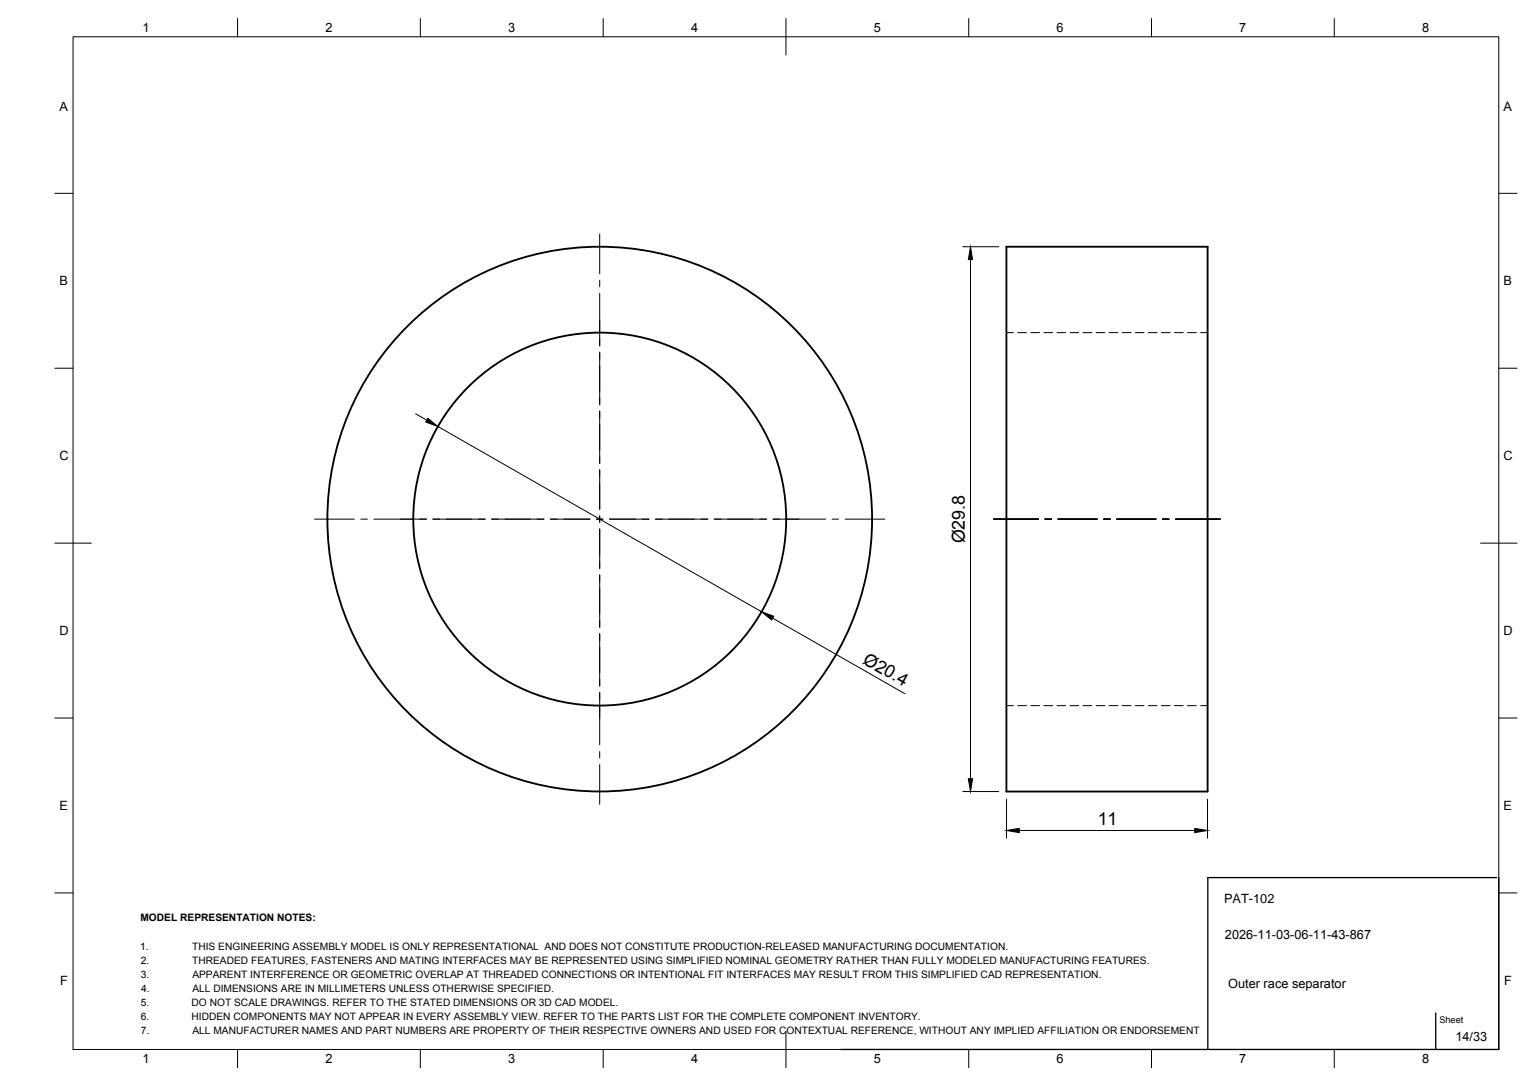
ISO-10303-21;
HEADER;
/* Generated by software containing ST-Developer
 * from STEP Tools, Inc. (www.steptools.com) 
 */

FILE_DESCRIPTION(
/* description */ ('Swing-away clamp arm'),
/* implementation_level */ '2;1');

FILE_NAME(
/* name */ 'Outer race separator.step',
/* time_stamp */ '2026-10-28T03:26:03-07:00',
/* author */ (''),
/* organization */ (''),
/* preprocessor_version */ 'ST-DEVELOPER v20.2',
/* originating_system */ 'Autodesk Translation Framework v15.17.0.0',
/* authorisation */ '');

FILE_SCHEMA (('AUTOMOTIVE_DESIGN { 1 0 10303 214 3 1 1 }'));
ENDSEC;

DATA;
#10=MECHANICAL_DESIGN_GEOMETRIC_PRESENTATION_REPRESENTATION('',(#301),#10627);
#249=SHAPE_REPRESENTATION_RELATIONSHIP('SRR','None',#10748,#275);
#275=ADVANCED_BREP_SHAPE_REPRESENTATION('',(#334),#10607);
#301=STYLED_ITEM('',(#10965),#334);
#334=MANIFOLD_SOLID_BREP('Body1',#4908);
#397=FACE_BOUND('',#1117,.T.);
#398=FACE_BOUND('',#1119,.T.);
#552=PLANE('',#5467);
#553=PLANE('',#5468);
#768=FACE_OUTER_BOUND('',#1114,.T.);
#769=FACE_OUTER_BOUND('',#1115,.T.);
#770=FACE_OUTER_BOUND('',#1116,.T.);
#771=FACE_OUTER_BOUND('',#1118,.T.);
#1114=EDGE_LOOP('',(#3849,#3850,#3851,#3852));
#1115=EDGE_LOOP('',(#3853,#3854,#3855,#3856));
#1116=EDGE_LOOP('',(#3857));
#1117=EDGE_LOOP('',(#3858));
#1118=EDGE_LOOP('',(#3859));
#1119=EDGE_LOOP('',(#3860));
#1548=LINE('',#9455,#1870);
#1549=LINE('',#9461,#1871);
#1870=VECTOR('',#6547,1.02);
#1871=VECTOR('',#6554,1.49);
#2081=CIRCLE('',#5462,1.02);
#2082=CIRCLE('',#5463,1.02);
#2083=CIRCLE('',#5465,1.49);
#2084=CIRCLE('',#5466,1.49);
#2450=VERTEX_POINT('',#9452);
#2451=VERTEX_POINT('',#9454);
#2452=VERTEX_POINT('',#9458);
#2453=VERTEX_POINT('',#9460);
#2957=EDGE_CURVE('',#2450,#2450,#2081,.T.);
#2958=EDGE_CURVE('',#2450,#2451,#1548,.T.);
#2959=EDGE_CURVE('',#2451,#2451,#2082,.T.);
#2960=EDGE_CURVE('',#2452,#2452,#2083,.T.);
#2961=EDGE_CURVE('',#2452,#2453,#1549,.T.);
#2962=EDGE_CURVE('',#2453,#2453,#2084,.T.);
#3849=ORIENTED_EDGE('',*,*,#2957,.F.);
#3850=ORIENTED_EDGE('',*,*,#2958,.T.);
#3851=ORIENTED_EDGE('',*,*,#2959,.T.);
#3852=ORIENTED_EDGE('',*,*,#2958,.F.);
#3853=ORIENTED_EDGE('',*,*,#2960,.F.);
#3854=ORIENTED_EDGE('',*,*,#2961,.T.);
#3855=ORIENTED_EDGE('',*,*,#2962,.T.);
#3856=ORIENTED_EDGE('',*,*,#2961,.F.);
#3857=ORIENTED_EDGE('',*,*,#2960,.T.);
#3858=ORIENTED_EDGE('',*,*,#2957,.T.);
#3859=ORIENTED_EDGE('',*,*,#2962,.F.);
#3860=ORIENTED_EDGE('',*,*,#2959,.F.);
#4530=CYLINDRICAL_SURFACE('',#5461,1.02);
#4531=CYLINDRICAL_SURFACE('',#5464,1.49);
#4723=ADVANCED_FACE('',(#768),#4530,.F.);
#4724=ADVANCED_FACE('',(#769),#4531,.T.);
#4725=ADVANCED_FACE('',(#770,#397),#552,.T.);
#4726=ADVANCED_FACE('',(#771,#398),#553,.F.);
#4908=CLOSED_SHELL('',(#4723,#4724,#4725,#4726));
#5460=AXIS2_PLACEMENT_3D('',#9450,#6541,#6542);
#5461=AXIS2_PLACEMENT_3D('',#9451,#6543,#6544);
#5462=AXIS2_PLACEMENT_3D('',#9453,#6545,#6546);
#5463=AXIS2_PLACEMENT_3D('',#9456,#6548,#6549);
#5464=AXIS2_PLACEMENT_3D('',#9457,#6550,#6551);
#5465=AXIS2_PLACEMENT_3D('',#9459,#6552,#6553);
#5466=AXIS2_PLACEMENT_3D('',#9462,#6555,#6556);
#5467=AXIS2_PLACEMENT_3D('',#9463,#6557,#6558);
#5468=AXIS2_PLACEMENT_3D('',#9464,#6559,#6560);
#6541=DIRECTION('axis',(0.,0.,1.));
#6542=DIRECTION('refdir',(1.,0.,0.));
#6543=DIRECTION('center_axis',(0.,0.,1.));
#6544=DIRECTION('ref_axis',(1.,0.,0.));
#6545=DIRECTION('center_axis',(0.,0.,-1.));
#6546=DIRECTION('ref_axis',(1.,0.,0.));
#6547=DIRECTION('',(0.,0.,-1.));
#6548=DIRECTION('center_axis',(0.,0.,-1.));
#6549=DIRECTION('ref_axis',(1.,0.,0.));
#6550=DIRECTION('center_axis',(0.,0.,1.));
#6551=DIRECTION('ref_axis',(1.,0.,0.));
#6552=DIRECTION('center_axis',(0.,0.,1.));
#6553=DIRECTION('ref_axis',(1.,0.,0.));
#6554=DIRECTION('',(0.,0.,-1.));
#6555=DIRECTION('center_axis',(0.,0.,1.));
#6556=DIRECTION('ref_axis',(1.,0.,0.));
#6557=DIRECTION('center_axis',(0.,0.,1.));
#6558=DIRECTION('ref_axis',(1.,0.,0.));
#6559=DIRECTION('center_axis',(0.,0.,1.));
#6560=DIRECTION('ref_axis',(1.,0.,0.));
#9450=CARTESIAN_POINT('',(0.,0.,0.));
#9451=CARTESIAN_POINT('Origin',(0.,0.,6.95));
#9452=CARTESIAN_POINT('',(-1.02,-1.2491397351303E-16,8.05));
#9453=CARTESIAN_POINT('Origin',(0.,0.,8.05));
#9454=CARTESIAN_POINT('',(-1.02,-1.2491397351303E-16,6.95));
#9455=CARTESIAN_POINT('',(-1.02,-1.2491397351303E-16,6.95));
#9456=CARTESIAN_POINT('Origin',(0.,0.,6.95));
#9457=CARTESIAN_POINT('Origin',(0.,0.,6.95));
#9458=CARTESIAN_POINT('',(-1.49,-1.82472373072956E-16,8.05));
#9459=CARTESIAN_POINT('Origin',(0.,0.,8.05));
#9460=CARTESIAN_POINT('',(-1.49,-1.82472373072956E-16,6.95));
#9461=CARTESIAN_POINT('',(-1.49,-1.82472373072956E-16,6.95));
#9462=CARTESIAN_POINT('Origin',(0.,0.,6.95));
#9463=CARTESIAN_POINT('Origin',(0.,0.,8.05));
#9464=CARTESIAN_POINT('Origin',(0.,0.,6.95));
#10575=UNCERTAINTY_MEASURE_WITH_UNIT(LENGTH_MEASURE(0.001),#10628,
'DISTANCE_ACCURACY_VALUE',
'Maximum model space distance between geometric entities at asserted c
onnectivities');
#10595=UNCERTAINTY_MEASURE_WITH_UNIT(LENGTH_MEASURE(0.001),#10628,
'DISTANCE_ACCURACY_VALUE',
'Maximum model space distance between geometric entities at asserted c
onnectivities');
#10607=(
GEOMETRIC_REPRESENTATION_CONTEXT(3)
GLOBAL_UNCERTAINTY_ASSIGNED_CONTEXT((#10575))
GLOBAL_UNIT_ASSIGNED_CONTEXT((#10628,#10630,#10631))
REPRESENTATION_CONTEXT('','3D')
);
#10627=(
GEOMETRIC_REPRESENTATION_CONTEXT(3)
GLOBAL_UNCERTAINTY_ASSIGNED_CONTEXT((#10595))
GLOBAL_UNIT_ASSIGNED_CONTEXT((#10628,#10630,#10631))
REPRESENTATION_CONTEXT('','3D')
);
#10628=(
LENGTH_UNIT()
NAMED_UNIT(*)
SI_UNIT(.CENTI.,.METRE.)
);
#10630=(
NAMED_UNIT(*)
PLANE_ANGLE_UNIT()
SI_UNIT($,.RADIAN.)
);
#10631=(
NAMED_UNIT(*)
SI_UNIT($,.STERADIAN.)
SOLID_ANGLE_UNIT()
);
#10643=SHAPE_DEFINITION_REPRESENTATION(#10684,#10748);
#10684=PRODUCT_DEFINITION_SHAPE('',$,#10780);
#10748=SHAPE_REPRESENTATION('',(#5460),#10607);
#10768=PRODUCT_DEFINITION_CONTEXT('part definition',#10863,'design');
#10780=PRODUCT_DEFINITION('Outer race separator','Outer race separator',
#10811,#10768);
#10811=PRODUCT_DEFINITION_FORMATION('',$,#10876);
#10863=APPLICATION_CONTEXT(
'Core Data for Automotive Mechanical Design Process');
#10864=PRODUCT_CONTEXT('part definition',#10863,'mechanical');
#10876=PRODUCT('Outer race separator','Outer race separator',
'Outer race separator',(#10864));
#10959=COLOUR_RGB('Grey',0.48,0.52,0.57);
#10960=FILL_AREA_STYLE_COLOUR('',#10959);
#10961=FILL_AREA_STYLE('',(#10960));
#10962=SURFACE_STYLE_FILL_AREA(#10961);
#10963=SURFACE_SIDE_STYLE('',(#10962));
#10964=SURFACE_STYLE_USAGE(.BOTH.,#10963);
#10965=PRESENTATION_STYLE_ASSIGNMENT((#10964));
ENDSEC;
END-ISO-10303-21;
